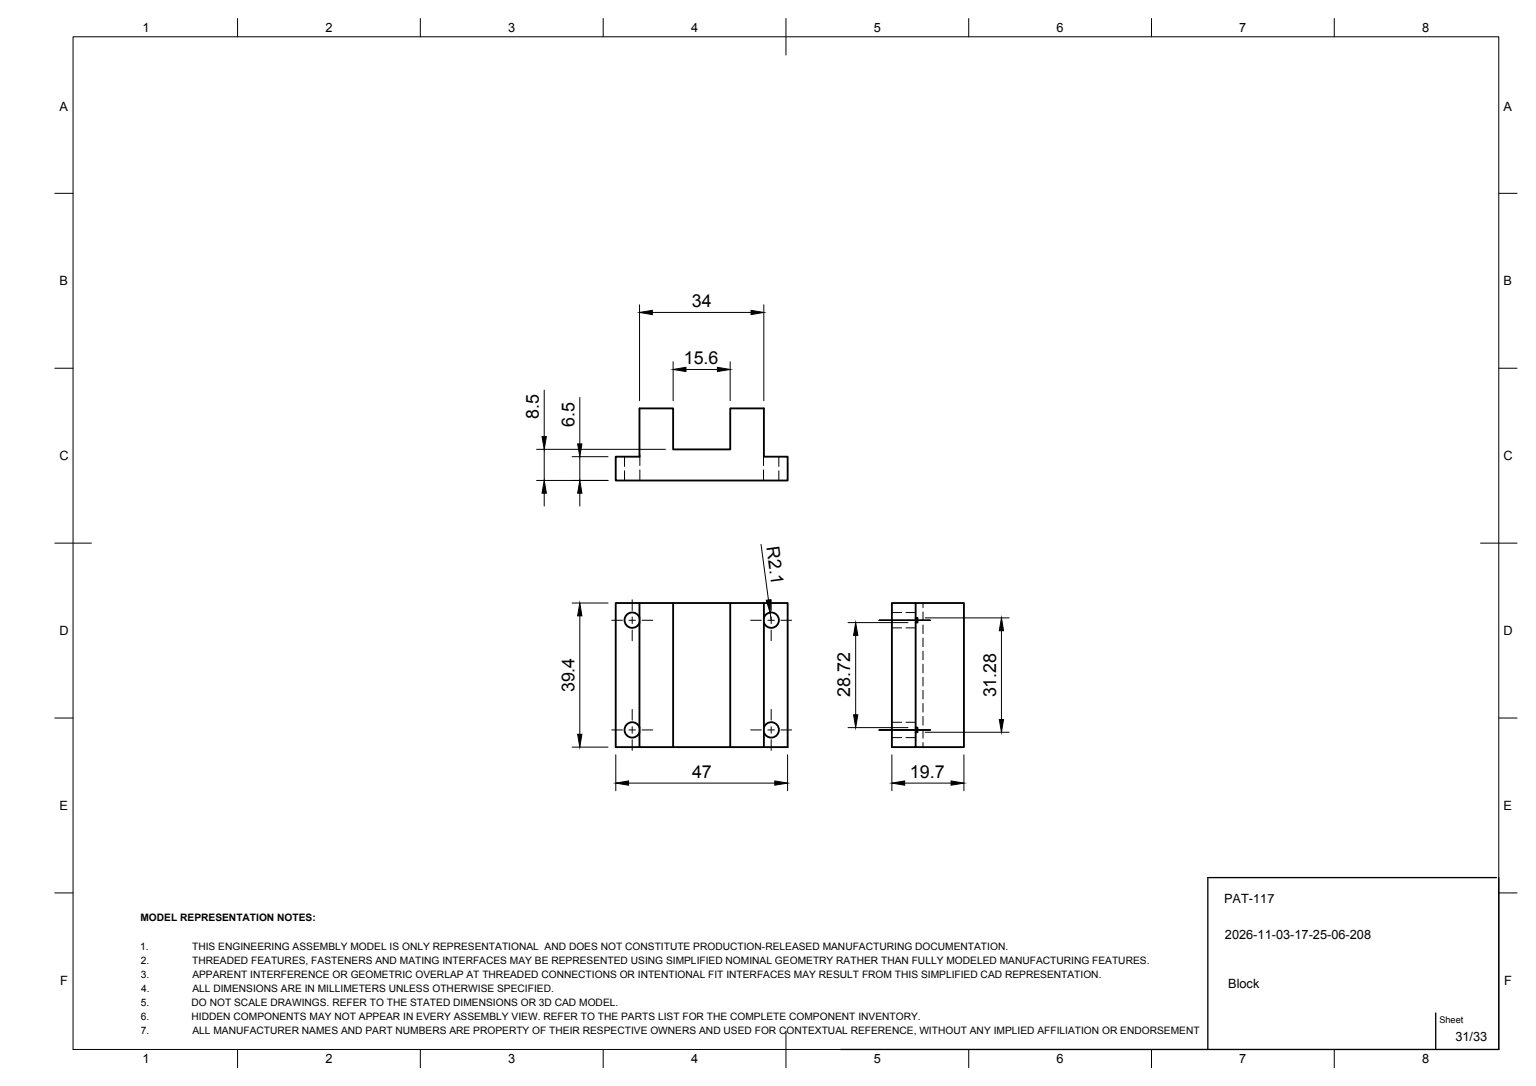
ISO-10303-21;
HEADER;
/* Generated by software containing ST-Developer
 * from STEP Tools, Inc. (www.steptools.com) 
 */

FILE_DESCRIPTION(
/* description */ ('Counterbalanced vertical column'),
/* implementation_level */ '2;1');

FILE_NAME(
/* name */ 'Block.step',
/* time_stamp */ '2026-10-29T16:47:22-07:00',
/* author */ (''),
/* organization */ (''),
/* preprocessor_version */ 'ST-DEVELOPER v20.2',
/* originating_system */ 'Autodesk Translation Framework v15.17.0.0',
/* authorisation */ '');

FILE_SCHEMA (('AUTOMOTIVE_DESIGN { 1 0 10303 214 3 1 1 }'));
ENDSEC;

DATA;
#10=MECHANICAL_DESIGN_GEOMETRIC_PRESENTATION_REPRESENTATION('',(#380),#15040);
#310=SHAPE_REPRESENTATION_RELATIONSHIP('SRR','None',#15216,#345);
#345=ADVANCED_BREP_SHAPE_REPRESENTATION('',(#413),#15035);
#380=STYLED_ITEM('',(#15436),#413);
#413=MANIFOLD_SOLID_BREP('Body1',#7105);
#525=FACE_BOUND('',#1684,.T.);
#526=FACE_BOUND('',#1685,.T.);
#527=FACE_BOUND('',#1686,.T.);
#528=FACE_BOUND('',#1687,.T.);
#766=PLANE('',#8052);
#767=PLANE('',#8058);
#768=PLANE('',#8064);
#769=PLANE('',#8070);
#770=PLANE('',#8076);
#771=PLANE('',#8077);
#772=PLANE('',#8078);
#773=PLANE('',#8079);
#774=PLANE('',#8080);
#775=PLANE('',#8081);
#776=PLANE('',#8082);
#777=PLANE('',#8083);
#778=PLANE('',#8084);
#779=PLANE('',#8085);
#780=PLANE('',#8086);
#781=PLANE('',#8087);
#782=PLANE('',#8088);
#783=PLANE('',#8089);
#1156=FACE_OUTER_BOUND('',#1670,.T.);
#1157=FACE_OUTER_BOUND('',#1671,.T.);
#1158=FACE_OUTER_BOUND('',#1672,.T.);
#1159=FACE_OUTER_BOUND('',#1673,.T.);
#1160=FACE_OUTER_BOUND('',#1674,.T.);
#1161=FACE_OUTER_BOUND('',#1675,.T.);
#1162=FACE_OUTER_BOUND('',#1676,.T.);
#1163=FACE_OUTER_BOUND('',#1677,.T.);
#1164=FACE_OUTER_BOUND('',#1678,.T.);
#1165=FACE_OUTER_BOUND('',#1679,.T.);
#1166=FACE_OUTER_BOUND('',#1680,.T.);
#1167=FACE_OUTER_BOUND('',#1681,.T.);
#1168=FACE_OUTER_BOUND('',#1682,.T.);
#1169=FACE_OUTER_BOUND('',#1683,.T.);
#1170=FACE_OUTER_BOUND('',#1688,.T.);
#1171=FACE_OUTER_BOUND('',#1689,.T.);
#1172=FACE_OUTER_BOUND('',#1690,.T.);
#1173=FACE_OUTER_BOUND('',#1691,.T.);
#1174=FACE_OUTER_BOUND('',#1692,.T.);
#1175=FACE_OUTER_BOUND('',#1693,.T.);
#1176=FACE_OUTER_BOUND('',#1694,.T.);
#1177=FACE_OUTER_BOUND('',#1695,.T.);
#1670=EDGE_LOOP('',(#6210,#6211));
#1671=EDGE_LOOP('',(#6212,#6213,#6214,#6215,#6216,#6217,#6218,#6219));
#1672=EDGE_LOOP('',(#6220,#6221));
#1673=EDGE_LOOP('',(#6222,#6223,#6224,#6225,#6226,#6227,#6228,#6229));
#1674=EDGE_LOOP('',(#6230,#6231));
#1675=EDGE_LOOP('',(#6232,#6233,#6234,#6235,#6236,#6237,#6238,#6239));
#1676=EDGE_LOOP('',(#6240,#6241));
#1677=EDGE_LOOP('',(#6242,#6243,#6244,#6245,#6246,#6247,#6248,#6249));
#1678=EDGE_LOOP('',(#6250,#6251,#6252,#6253,#6254,#6255,#6256,#6257,#6258,
#6259,#6260,#6261));
#1679=EDGE_LOOP('',(#6262,#6263,#6264,#6265,#6266,#6267,#6268,#6269,#6270,
#6271,#6272,#6273));
#1680=EDGE_LOOP('',(#6274,#6275,#6276,#6277,#6278,#6279,#6280,#6281,#6282,
#6283,#6284,#6285));
#1681=EDGE_LOOP('',(#6286,#6287,#6288,#6289,#6290,#6291,#6292,#6293,#6294,
#6295));
#1682=EDGE_LOOP('',(#6296,#6297,#6298,#6299));
#1683=EDGE_LOOP('',(#6300,#6301,#6302,#6303));
#1684=EDGE_LOOP('',(#6304));
#1685=EDGE_LOOP('',(#6305));
#1686=EDGE_LOOP('',(#6306));
#1687=EDGE_LOOP('',(#6307));
#1688=EDGE_LOOP('',(#6308,#6309,#6310,#6311));
#1689=EDGE_LOOP('',(#6312,#6313,#6314,#6315,#6316,#6317,#6318,#6319,#6320,
#6321));
#1690=EDGE_LOOP('',(#6322,#6323,#6324,#6325));
#1691=EDGE_LOOP('',(#6326,#6327,#6328,#6329));
#1692=EDGE_LOOP('',(#6330,#6331,#6332,#6333));
#1693=EDGE_LOOP('',(#6334,#6335,#6336,#6337));
#1694=EDGE_LOOP('',(#6338,#6339,#6340,#6341));
#1695=EDGE_LOOP('',(#6342,#6343,#6344,#6345,#6346,#6347,#6348,#6349,#6350,
#6351,#6352,#6353));
#2271=LINE('',#14525,#2942);
#2272=LINE('',#14529,#2943);
#2273=LINE('',#14533,#2944);
#2274=LINE('',#14537,#2945);
#2275=LINE('',#14541,#2946);
#2276=LINE('',#14545,#2947);
#2277=LINE('',#14549,#2948);
#2278=LINE('',#14553,#2949);
#2279=LINE('',#14557,#2950);
#2280=LINE('',#14561,#2951);
#2281=LINE('',#14565,#2952);
#2282=LINE('',#14569,#2953);
#2283=LINE('',#14573,#2954);
#2284=LINE('',#14577,#2955);
#2285=LINE('',#14581,#2956);
#2286=LINE('',#14585,#2957);
#2287=LINE('',#14587,#2958);
#2288=LINE('',#14589,#2959);
#2289=LINE('',#14591,#2960);
#2290=LINE('',#14593,#2961);
#2291=LINE('',#14595,#2962);
#2292=LINE('',#14596,#2963);
#2293=LINE('',#14598,#2964);
#2294=LINE('',#14600,#2965);
#2295=LINE('',#14602,#2966);
#2296=LINE('',#14604,#2967);
#2297=LINE('',#14606,#2968);
#2298=LINE('',#14607,#2969);
#2299=LINE('',#14610,#2970);
#2300=LINE('',#14612,#2971);
#2301=LINE('',#14614,#2972);
#2302=LINE('',#14616,#2973);
#2303=LINE('',#14617,#2974);
#2304=LINE('',#14619,#2975);
#2305=LINE('',#14621,#2976);
#2306=LINE('',#14623,#2977);
#2307=LINE('',#14625,#2978);
#2308=LINE('',#14626,#2979);
#2309=LINE('',#14629,#2980);
#2310=LINE('',#14630,#2981);
#2311=LINE('',#14633,#2982);
#2312=LINE('',#14634,#2983);
#2313=LINE('',#14637,#2984);
#2314=LINE('',#14638,#2985);
#2315=LINE('',#14641,#2986);
#2316=LINE('',#14642,#2987);
#2317=LINE('',#14644,#2988);
#2318=LINE('',#14647,#2989);
#2319=LINE('',#14648,#2990);
#2320=LINE('',#14651,#2991);
#2321=LINE('',#14652,#2992);
#2322=LINE('',#14655,#2993);
#2323=LINE('',#14656,#2994);
#2324=LINE('',#14659,#2995);
#2325=LINE('',#14660,#2996);
#2326=LINE('',#14662,#2997);
#2942=VECTOR('',#9851,1.);
#2943=VECTOR('',#9856,1.);
#2944=VECTOR('',#9859,0.21);
#2945=VECTOR('',#9864,1.);
#2946=VECTOR('',#9867,1.);
#2947=VECTOR('',#9872,1.);
#2948=VECTOR('',#9875,0.21);
#2949=VECTOR('',#9880,1.);
#2950=VECTOR('',#9883,1.);
#2951=VECTOR('',#9888,1.);
#2952=VECTOR('',#9891,0.21);
#2953=VECTOR('',#9896,1.);
#2954=VECTOR('',#9899,1.);
#2955=VECTOR('',#9904,1.);
#2956=VECTOR('',#9907,0.21);
#2957=VECTOR('',#9912,1.);
#2958=VECTOR('',#9915,1.);
#2959=VECTOR('',#9916,1.);
#2960=VECTOR('',#9917,1.);
#2961=VECTOR('',#9918,1.);
#2962=VECTOR('',#9919,1.);
#2963=VECTOR('',#9920,1.);
#2964=VECTOR('',#9923,1.);
#2965=VECTOR('',#9924,1.);
#2966=VECTOR('',#9925,1.);
#2967=VECTOR('',#9926,1.);
#2968=VECTOR('',#9927,1.);
#2969=VECTOR('',#9928,1.);
#2970=VECTOR('',#9931,1.);
#2971=VECTOR('',#9932,1.);
#2972=VECTOR('',#9933,1.);
#2973=VECTOR('',#9934,1.);
#2974=VECTOR('',#9935,1.);
#2975=VECTOR('',#9936,1.);
#2976=VECTOR('',#9937,1.);
#2977=VECTOR('',#9938,1.);
#2978=VECTOR('',#9939,1.);
#2979=VECTOR('',#9940,1.);
#2980=VECTOR('',#9943,1.);
#2981=VECTOR('',#9944,1.);
#2982=VECTOR('',#9947,1.);
#2983=VECTOR('',#9948,1.);
#2984=VECTOR('',#9951,1.);
#2985=VECTOR('',#9952,1.);
#2986=VECTOR('',#9955,1.);
#2987=VECTOR('',#9956,1.);
#2988=VECTOR('',#9959,1.);
#2989=VECTOR('',#9962,1.);
#2990=VECTOR('',#9963,1.);
#2991=VECTOR('',#9966,1.);
#2992=VECTOR('',#9967,1.);
#2993=VECTOR('',#9970,1.);
#2994=VECTOR('',#9971,1.);
#2995=VECTOR('',#9974,1.);
#2996=VECTOR('',#9975,1.);
#2997=VECTOR('',#9978,1.);
#3275=CIRCLE('',#8053,0.21);
#3276=CIRCLE('',#8055,0.21);
#3277=CIRCLE('',#8056,0.21);
#3278=CIRCLE('',#8057,0.21);
#3279=CIRCLE('',#8059,0.21);
#3280=CIRCLE('',#8061,0.21);
#3281=CIRCLE('',#8062,0.21);
#3282=CIRCLE('',#8063,0.21);
#3283=CIRCLE('',#8065,0.21);
#3284=CIRCLE('',#8067,0.21);
#3285=CIRCLE('',#8068,0.21);
#3286=CIRCLE('',#8069,0.21);
#3287=CIRCLE('',#8071,0.21);
#3288=CIRCLE('',#8073,0.21);
#3289=CIRCLE('',#8074,0.21);
#3290=CIRCLE('',#8075,0.21);
#3776=VERTEX_POINT('',#14523);
#3777=VERTEX_POINT('',#14524);
#3778=VERTEX_POINT('',#14528);
#3779=VERTEX_POINT('',#14530);
#3780=VERTEX_POINT('',#14532);
#3781=VERTEX_POINT('',#14535);
#3782=VERTEX_POINT('',#14539);
#3783=VERTEX_POINT('',#14540);
#3784=VERTEX_POINT('',#14544);
#3785=VERTEX_POINT('',#14546);
#3786=VERTEX_POINT('',#14548);
#3787=VERTEX_POINT('',#14551);
#3788=VERTEX_POINT('',#14555);
#3789=VERTEX_POINT('',#14556);
#3790=VERTEX_POINT('',#14560);
#3791=VERTEX_POINT('',#14562);
#3792=VERTEX_POINT('',#14564);
#3793=VERTEX_POINT('',#14567);
#3794=VERTEX_POINT('',#14571);
#3795=VERTEX_POINT('',#14572);
#3796=VERTEX_POINT('',#14576);
#3797=VERTEX_POINT('',#14578);
#3798=VERTEX_POINT('',#14580);
#3799=VERTEX_POINT('',#14583);
#3800=VERTEX_POINT('',#14588);
#3801=VERTEX_POINT('',#14590);
#3802=VERTEX_POINT('',#14592);
#3803=VERTEX_POINT('',#14594);
#3804=VERTEX_POINT('',#14599);
#3805=VERTEX_POINT('',#14601);
#3806=VERTEX_POINT('',#14603);
#3807=VERTEX_POINT('',#14605);
#3808=VERTEX_POINT('',#14609);
#3809=VERTEX_POINT('',#14611);
#3810=VERTEX_POINT('',#14613);
#3811=VERTEX_POINT('',#14615);
#3812=VERTEX_POINT('',#14618);
#3813=VERTEX_POINT('',#14620);
#3814=VERTEX_POINT('',#14622);
#3815=VERTEX_POINT('',#14624);
#3816=VERTEX_POINT('',#14628);
#3817=VERTEX_POINT('',#14632);
#3818=VERTEX_POINT('',#14636);
#3819=VERTEX_POINT('',#14640);
#3820=VERTEX_POINT('',#14646);
#3821=VERTEX_POINT('',#14650);
#3822=VERTEX_POINT('',#14654);
#3823=VERTEX_POINT('',#14658);
#4606=EDGE_CURVE('',#3776,#3777,#2271,.T.);
#4607=EDGE_CURVE('',#3776,#3777,#3275,.T.);
#4608=EDGE_CURVE('',#3778,#3776,#2272,.T.);
#4609=EDGE_CURVE('',#3779,#3778,#3276,.T.);
#4610=EDGE_CURVE('',#3779,#3780,#2273,.T.);
#4611=EDGE_CURVE('',#3780,#3780,#3277,.T.);
#4612=EDGE_CURVE('',#3781,#3779,#3278,.T.);
#4613=EDGE_CURVE('',#3777,#3781,#2274,.T.);
#4614=EDGE_CURVE('',#3782,#3783,#2275,.T.);
#4615=EDGE_CURVE('',#3782,#3783,#3279,.T.);
#4616=EDGE_CURVE('',#3784,#3782,#2276,.T.);
#4617=EDGE_CURVE('',#3785,#3784,#3280,.T.);
#4618=EDGE_CURVE('',#3785,#3786,#2277,.T.);
#4619=EDGE_CURVE('',#3786,#3786,#3281,.T.);
#4620=EDGE_CURVE('',#3787,#3785,#3282,.T.);
#4621=EDGE_CURVE('',#3783,#3787,#2278,.T.);
#4622=EDGE_CURVE('',#3788,#3789,#2279,.T.);
#4623=EDGE_CURVE('',#3788,#3789,#3283,.T.);
#4624=EDGE_CURVE('',#3790,#3788,#2280,.T.);
#4625=EDGE_CURVE('',#3791,#3790,#3284,.T.);
#4626=EDGE_CURVE('',#3791,#3792,#2281,.T.);
#4627=EDGE_CURVE('',#3792,#3792,#3285,.T.);
#4628=EDGE_CURVE('',#3793,#3791,#3286,.T.);
#4629=EDGE_CURVE('',#3789,#3793,#2282,.T.);
#4630=EDGE_CURVE('',#3794,#3795,#2283,.T.);
#4631=EDGE_CURVE('',#3794,#3795,#3287,.T.);
#4632=EDGE_CURVE('',#3796,#3794,#2284,.T.);
#4633=EDGE_CURVE('',#3797,#3796,#3288,.T.);
#4634=EDGE_CURVE('',#3797,#3798,#2285,.T.);
#4635=EDGE_CURVE('',#3798,#3798,#3289,.T.);
#4636=EDGE_CURVE('',#3799,#3797,#3290,.T.);
#4637=EDGE_CURVE('',#3795,#3799,#2286,.T.);
#4638=EDGE_CURVE('',#3781,#3790,#2287,.T.);
#4639=EDGE_CURVE('',#3793,#3800,#2288,.T.);
#4640=EDGE_CURVE('',#3801,#3800,#2289,.T.);
#4641=EDGE_CURVE('',#3801,#3802,#2290,.T.);
#4642=EDGE_CURVE('',#3803,#3802,#2291,.T.);
#4643=EDGE_CURVE('',#3803,#3778,#2292,.T.);
#4644=EDGE_CURVE('',#3787,#3796,#2293,.T.);
#4645=EDGE_CURVE('',#3799,#3804,#2294,.T.);
#4646=EDGE_CURVE('',#3805,#3804,#2295,.T.);
#4647=EDGE_CURVE('',#3806,#3805,#2296,.T.);
#4648=EDGE_CURVE('',#3807,#3806,#2297,.T.);
#4649=EDGE_CURVE('',#3807,#3784,#2298,.T.);
#4650=EDGE_CURVE('',#3800,#3808,#2299,.T.);
#4651=EDGE_CURVE('',#3808,#3809,#2300,.T.);
#4652=EDGE_CURVE('',#3809,#3810,#2301,.T.);
#4653=EDGE_CURVE('',#3810,#3811,#2302,.T.);
#4654=EDGE_CURVE('',#3811,#3807,#2303,.T.);
#4655=EDGE_CURVE('',#3806,#3812,#2304,.T.);
#4656=EDGE_CURVE('',#3812,#3813,#2305,.T.);
#4657=EDGE_CURVE('',#3813,#3814,#2306,.T.);
#4658=EDGE_CURVE('',#3814,#3815,#2307,.T.);
#4659=EDGE_CURVE('',#3815,#3801,#2308,.T.);
#4660=EDGE_CURVE('',#3816,#3803,#2309,.T.);
#4661=EDGE_CURVE('',#3808,#3816,#2310,.T.);
#4662=EDGE_CURVE('',#3817,#3816,#2311,.T.);
#4663=EDGE_CURVE('',#3809,#3817,#2312,.T.);
#4664=EDGE_CURVE('',#3818,#3817,#2313,.T.);
#4665=EDGE_CURVE('',#3810,#3818,#2314,.T.);
#4666=EDGE_CURVE('',#3819,#3818,#2315,.T.);
#4667=EDGE_CURVE('',#3811,#3819,#2316,.T.);
#4668=EDGE_CURVE('',#3804,#3819,#2317,.T.);
#4669=EDGE_CURVE('',#3820,#3805,#2318,.T.);
#4670=EDGE_CURVE('',#3812,#3820,#2319,.T.);
#4671=EDGE_CURVE('',#3821,#3820,#2320,.T.);
#4672=EDGE_CURVE('',#3813,#3821,#2321,.T.);
#4673=EDGE_CURVE('',#3822,#3821,#2322,.T.);
#4674=EDGE_CURVE('',#3814,#3822,#2323,.T.);
#4675=EDGE_CURVE('',#3823,#3822,#2324,.T.);
#4676=EDGE_CURVE('',#3815,#3823,#2325,.T.);
#4677=EDGE_CURVE('',#3802,#3823,#2326,.T.);
#6210=ORIENTED_EDGE('',*,*,#4606,.F.);
#6211=ORIENTED_EDGE('',*,*,#4607,.T.);
#6212=ORIENTED_EDGE('',*,*,#4608,.F.);
#6213=ORIENTED_EDGE('',*,*,#4609,.F.);
#6214=ORIENTED_EDGE('',*,*,#4610,.T.);
#6215=ORIENTED_EDGE('',*,*,#4611,.F.);
#6216=ORIENTED_EDGE('',*,*,#4610,.F.);
#6217=ORIENTED_EDGE('',*,*,#4612,.F.);
#6218=ORIENTED_EDGE('',*,*,#4613,.F.);
#6219=ORIENTED_EDGE('',*,*,#4607,.F.);
#6220=ORIENTED_EDGE('',*,*,#4614,.F.);
#6221=ORIENTED_EDGE('',*,*,#4615,.T.);
#6222=ORIENTED_EDGE('',*,*,#4616,.F.);
#6223=ORIENTED_EDGE('',*,*,#4617,.F.);
#6224=ORIENTED_EDGE('',*,*,#4618,.T.);
#6225=ORIENTED_EDGE('',*,*,#4619,.F.);
#6226=ORIENTED_EDGE('',*,*,#4618,.F.);
#6227=ORIENTED_EDGE('',*,*,#4620,.F.);
#6228=ORIENTED_EDGE('',*,*,#4621,.F.);
#6229=ORIENTED_EDGE('',*,*,#4615,.F.);
#6230=ORIENTED_EDGE('',*,*,#4622,.F.);
#6231=ORIENTED_EDGE('',*,*,#4623,.T.);
#6232=ORIENTED_EDGE('',*,*,#4624,.F.);
#6233=ORIENTED_EDGE('',*,*,#4625,.F.);
#6234=ORIENTED_EDGE('',*,*,#4626,.T.);
#6235=ORIENTED_EDGE('',*,*,#4627,.F.);
#6236=ORIENTED_EDGE('',*,*,#4626,.F.);
#6237=ORIENTED_EDGE('',*,*,#4628,.F.);
#6238=ORIENTED_EDGE('',*,*,#4629,.F.);
#6239=ORIENTED_EDGE('',*,*,#4623,.F.);
#6240=ORIENTED_EDGE('',*,*,#4630,.F.);
#6241=ORIENTED_EDGE('',*,*,#4631,.T.);
#6242=ORIENTED_EDGE('',*,*,#4632,.F.);
#6243=ORIENTED_EDGE('',*,*,#4633,.F.);
#6244=ORIENTED_EDGE('',*,*,#4634,.T.);
#6245=ORIENTED_EDGE('',*,*,#4635,.F.);
#6246=ORIENTED_EDGE('',*,*,#4634,.F.);
#6247=ORIENTED_EDGE('',*,*,#4636,.F.);
#6248=ORIENTED_EDGE('',*,*,#4637,.F.);
#6249=ORIENTED_EDGE('',*,*,#4631,.F.);
#6250=ORIENTED_EDGE('',*,*,#4608,.T.);
#6251=ORIENTED_EDGE('',*,*,#4606,.T.);
#6252=ORIENTED_EDGE('',*,*,#4613,.T.);
#6253=ORIENTED_EDGE('',*,*,#4638,.T.);
#6254=ORIENTED_EDGE('',*,*,#4624,.T.);
#6255=ORIENTED_EDGE('',*,*,#4622,.T.);
#6256=ORIENTED_EDGE('',*,*,#4629,.T.);
#6257=ORIENTED_EDGE('',*,*,#4639,.T.);
#6258=ORIENTED_EDGE('',*,*,#4640,.F.);
#6259=ORIENTED_EDGE('',*,*,#4641,.T.);
#6260=ORIENTED_EDGE('',*,*,#4642,.F.);
#6261=ORIENTED_EDGE('',*,*,#4643,.T.);
#6262=ORIENTED_EDGE('',*,*,#4616,.T.);
#6263=ORIENTED_EDGE('',*,*,#4614,.T.);
#6264=ORIENTED_EDGE('',*,*,#4621,.T.);
#6265=ORIENTED_EDGE('',*,*,#4644,.T.);
#6266=ORIENTED_EDGE('',*,*,#4632,.T.);
#6267=ORIENTED_EDGE('',*,*,#4630,.T.);
#6268=ORIENTED_EDGE('',*,*,#4637,.T.);
#6269=ORIENTED_EDGE('',*,*,#4645,.T.);
#6270=ORIENTED_EDGE('',*,*,#4646,.F.);
#6271=ORIENTED_EDGE('',*,*,#4647,.F.);
#6272=ORIENTED_EDGE('',*,*,#4648,.F.);
#6273=ORIENTED_EDGE('',*,*,#4649,.T.);
#6274=ORIENTED_EDGE('',*,*,#4640,.T.);
#6275=ORIENTED_EDGE('',*,*,#4650,.T.);
#6276=ORIENTED_EDGE('',*,*,#4651,.T.);
#6277=ORIENTED_EDGE('',*,*,#4652,.T.);
#6278=ORIENTED_EDGE('',*,*,#4653,.T.);
#6279=ORIENTED_EDGE('',*,*,#4654,.T.);
#6280=ORIENTED_EDGE('',*,*,#4648,.T.);
#6281=ORIENTED_EDGE('',*,*,#4655,.T.);
#6282=ORIENTED_EDGE('',*,*,#4656,.T.);
#6283=ORIENTED_EDGE('',*,*,#4657,.T.);
#6284=ORIENTED_EDGE('',*,*,#4658,.T.);
#6285=ORIENTED_EDGE('',*,*,#4659,.T.);
#6286=ORIENTED_EDGE('',*,*,#4612,.T.);
#6287=ORIENTED_EDGE('',*,*,#4609,.T.);
#6288=ORIENTED_EDGE('',*,*,#4643,.F.);
#6289=ORIENTED_EDGE('',*,*,#4660,.F.);
#6290=ORIENTED_EDGE('',*,*,#4661,.F.);
#6291=ORIENTED_EDGE('',*,*,#4650,.F.);
#6292=ORIENTED_EDGE('',*,*,#4639,.F.);
#6293=ORIENTED_EDGE('',*,*,#4628,.T.);
#6294=ORIENTED_EDGE('',*,*,#4625,.T.);
#6295=ORIENTED_EDGE('',*,*,#4638,.F.);
#6296=ORIENTED_EDGE('',*,*,#4661,.T.);
#6297=ORIENTED_EDGE('',*,*,#4662,.F.);
#6298=ORIENTED_EDGE('',*,*,#4663,.F.);
#6299=ORIENTED_EDGE('',*,*,#4651,.F.);
#6300=ORIENTED_EDGE('',*,*,#4663,.T.);
#6301=ORIENTED_EDGE('',*,*,#4664,.F.);
#6302=ORIENTED_EDGE('',*,*,#4665,.F.);
#6303=ORIENTED_EDGE('',*,*,#4652,.F.);
#6304=ORIENTED_EDGE('',*,*,#4611,.T.);
#6305=ORIENTED_EDGE('',*,*,#4619,.T.);
#6306=ORIENTED_EDGE('',*,*,#4627,.T.);
#6307=ORIENTED_EDGE('',*,*,#4635,.T.);
#6308=ORIENTED_EDGE('',*,*,#4665,.T.);
#6309=ORIENTED_EDGE('',*,*,#4666,.F.);
#6310=ORIENTED_EDGE('',*,*,#4667,.F.);
#6311=ORIENTED_EDGE('',*,*,#4653,.F.);
#6312=ORIENTED_EDGE('',*,*,#4620,.T.);
#6313=ORIENTED_EDGE('',*,*,#4617,.T.);
#6314=ORIENTED_EDGE('',*,*,#4649,.F.);
#6315=ORIENTED_EDGE('',*,*,#4654,.F.);
#6316=ORIENTED_EDGE('',*,*,#4667,.T.);
#6317=ORIENTED_EDGE('',*,*,#4668,.F.);
#6318=ORIENTED_EDGE('',*,*,#4645,.F.);
#6319=ORIENTED_EDGE('',*,*,#4636,.T.);
#6320=ORIENTED_EDGE('',*,*,#4633,.T.);
#6321=ORIENTED_EDGE('',*,*,#4644,.F.);
#6322=ORIENTED_EDGE('',*,*,#4647,.T.);
#6323=ORIENTED_EDGE('',*,*,#4669,.F.);
#6324=ORIENTED_EDGE('',*,*,#4670,.F.);
#6325=ORIENTED_EDGE('',*,*,#4655,.F.);
#6326=ORIENTED_EDGE('',*,*,#4670,.T.);
#6327=ORIENTED_EDGE('',*,*,#4671,.F.);
#6328=ORIENTED_EDGE('',*,*,#4672,.F.);
#6329=ORIENTED_EDGE('',*,*,#4656,.F.);
#6330=ORIENTED_EDGE('',*,*,#4672,.T.);
#6331=ORIENTED_EDGE('',*,*,#4673,.F.);
#6332=ORIENTED_EDGE('',*,*,#4674,.F.);
#6333=ORIENTED_EDGE('',*,*,#4657,.F.);
#6334=ORIENTED_EDGE('',*,*,#4674,.T.);
#6335=ORIENTED_EDGE('',*,*,#4675,.F.);
#6336=ORIENTED_EDGE('',*,*,#4676,.F.);
#6337=ORIENTED_EDGE('',*,*,#4658,.F.);
#6338=ORIENTED_EDGE('',*,*,#4676,.T.);
#6339=ORIENTED_EDGE('',*,*,#4677,.F.);
#6340=ORIENTED_EDGE('',*,*,#4641,.F.);
#6341=ORIENTED_EDGE('',*,*,#4659,.F.);
#6342=ORIENTED_EDGE('',*,*,#4642,.T.);
#6343=ORIENTED_EDGE('',*,*,#4677,.T.);
#6344=ORIENTED_EDGE('',*,*,#4675,.T.);
#6345=ORIENTED_EDGE('',*,*,#4673,.T.);
#6346=ORIENTED_EDGE('',*,*,#4671,.T.);
#6347=ORIENTED_EDGE('',*,*,#4669,.T.);
#6348=ORIENTED_EDGE('',*,*,#4646,.T.);
#6349=ORIENTED_EDGE('',*,*,#4668,.T.);
#6350=ORIENTED_EDGE('',*,*,#4666,.T.);
#6351=ORIENTED_EDGE('',*,*,#4664,.T.);
#6352=ORIENTED_EDGE('',*,*,#4662,.T.);
#6353=ORIENTED_EDGE('',*,*,#4660,.T.);
#6660=CYLINDRICAL_SURFACE('',#8054,0.21);
#6661=CYLINDRICAL_SURFACE('',#8060,0.21);
#6662=CYLINDRICAL_SURFACE('',#8066,0.21);
#6663=CYLINDRICAL_SURFACE('',#8072,0.21);
#6998=ADVANCED_FACE('',(#1156),#766,.T.);
#6999=ADVANCED_FACE('',(#1157),#6660,.F.);
#7000=ADVANCED_FACE('',(#1158),#767,.T.);
#7001=ADVANCED_FACE('',(#1159),#6661,.F.);
#7002=ADVANCED_FACE('',(#1160),#768,.T.);
#7003=ADVANCED_FACE('',(#1161),#6662,.F.);
#7004=ADVANCED_FACE('',(#1162),#769,.T.);
#7005=ADVANCED_FACE('',(#1163),#6663,.F.);
#7006=ADVANCED_FACE('',(#1164),#770,.T.);
#7007=ADVANCED_FACE('',(#1165),#771,.T.);
#7008=ADVANCED_FACE('',(#1166),#772,.T.);
#7009=ADVANCED_FACE('',(#1167),#773,.T.);
#7010=ADVANCED_FACE('',(#1168),#774,.T.);
#7011=ADVANCED_FACE('',(#1169,#525,#526,#527,#528),#775,.T.);
#7012=ADVANCED_FACE('',(#1170),#776,.T.);
#7013=ADVANCED_FACE('',(#1171),#777,.T.);
#7014=ADVANCED_FACE('',(#1172),#778,.T.);
#7015=ADVANCED_FACE('',(#1173),#779,.T.);
#7016=ADVANCED_FACE('',(#1174),#780,.T.);
#7017=ADVANCED_FACE('',(#1175),#781,.T.);
#7018=ADVANCED_FACE('',(#1176),#782,.T.);
#7019=ADVANCED_FACE('',(#1177),#783,.T.);
#7105=CLOSED_SHELL('',(#6998,#6999,#7000,#7001,#7002,#7003,#7004,#7005,
#7006,#7007,#7008,#7009,#7010,#7011,#7012,#7013,#7014,#7015,#7016,#7017,
#7018,#7019));
#8051=AXIS2_PLACEMENT_3D('',#14521,#9847,#9848);
#8052=AXIS2_PLACEMENT_3D('',#14522,#9849,#9850);
#8053=AXIS2_PLACEMENT_3D('',#14526,#9852,#9853);
#8054=AXIS2_PLACEMENT_3D('',#14527,#9854,#9855);
#8055=AXIS2_PLACEMENT_3D('',#14531,#9857,#9858);
#8056=AXIS2_PLACEMENT_3D('',#14534,#9860,#9861);
#8057=AXIS2_PLACEMENT_3D('',#14536,#9862,#9863);
#8058=AXIS2_PLACEMENT_3D('',#14538,#9865,#9866);
#8059=AXIS2_PLACEMENT_3D('',#14542,#9868,#9869);
#8060=AXIS2_PLACEMENT_3D('',#14543,#9870,#9871);
#8061=AXIS2_PLACEMENT_3D('',#14547,#9873,#9874);
#8062=AXIS2_PLACEMENT_3D('',#14550,#9876,#9877);
#8063=AXIS2_PLACEMENT_3D('',#14552,#9878,#9879);
#8064=AXIS2_PLACEMENT_3D('',#14554,#9881,#9882);
#8065=AXIS2_PLACEMENT_3D('',#14558,#9884,#9885);
#8066=AXIS2_PLACEMENT_3D('',#14559,#9886,#9887);
#8067=AXIS2_PLACEMENT_3D('',#14563,#9889,#9890);
#8068=AXIS2_PLACEMENT_3D('',#14566,#9892,#9893);
#8069=AXIS2_PLACEMENT_3D('',#14568,#9894,#9895);
#8070=AXIS2_PLACEMENT_3D('',#14570,#9897,#9898);
#8071=AXIS2_PLACEMENT_3D('',#14574,#9900,#9901);
#8072=AXIS2_PLACEMENT_3D('',#14575,#9902,#9903);
#8073=AXIS2_PLACEMENT_3D('',#14579,#9905,#9906);
#8074=AXIS2_PLACEMENT_3D('',#14582,#9908,#9909);
#8075=AXIS2_PLACEMENT_3D('',#14584,#9910,#9911);
#8076=AXIS2_PLACEMENT_3D('',#14586,#9913,#9914);
#8077=AXIS2_PLACEMENT_3D('',#14597,#9921,#9922);
#8078=AXIS2_PLACEMENT_3D('',#14608,#9929,#9930);
#8079=AXIS2_PLACEMENT_3D('',#14627,#9941,#9942);
#8080=AXIS2_PLACEMENT_3D('',#14631,#9945,#9946);
#8081=AXIS2_PLACEMENT_3D('',#14635,#9949,#9950);
#8082=AXIS2_PLACEMENT_3D('',#14639,#9953,#9954);
#8083=AXIS2_PLACEMENT_3D('',#14643,#9957,#9958);
#8084=AXIS2_PLACEMENT_3D('',#14645,#9960,#9961);
#8085=AXIS2_PLACEMENT_3D('',#14649,#9964,#9965);
#8086=AXIS2_PLACEMENT_3D('',#14653,#9968,#9969);
#8087=AXIS2_PLACEMENT_3D('',#14657,#9972,#9973);
#8088=AXIS2_PLACEMENT_3D('',#14661,#9976,#9977);
#8089=AXIS2_PLACEMENT_3D('',#14663,#9979,#9980);
#9847=DIRECTION('axis',(0.,0.,1.));
#9848=DIRECTION('refdir',(1.,0.,0.));
#9849=DIRECTION('center_axis',(0.,0.,1.));
#9850=DIRECTION('ref_axis',(1.,0.,0.));
#9851=DIRECTION('',(-1.,0.,0.));
#9852=DIRECTION('center_axis',(0.,0.,1.));
#9853=DIRECTION('ref_axis',(1.,0.,0.));
#9854=DIRECTION('center_axis',(0.,0.,1.));
#9855=DIRECTION('ref_axis',(1.,0.,0.));
#9856=DIRECTION('',(0.,0.,-1.));
#9857=DIRECTION('center_axis',(0.,0.,1.));
#9858=DIRECTION('ref_axis',(1.,0.,0.));
#9859=DIRECTION('',(0.,0.,1.));
#9860=DIRECTION('center_axis',(0.,0.,-1.));
#9861=DIRECTION('ref_axis',(1.,0.,0.));
#9862=DIRECTION('center_axis',(0.,0.,1.));
#9863=DIRECTION('ref_axis',(1.,0.,0.));
#9864=DIRECTION('',(0.,0.,1.));
#9865=DIRECTION('center_axis',(0.,0.,1.));
#9866=DIRECTION('ref_axis',(1.,0.,0.));
#9867=DIRECTION('',(1.,0.,0.));
#9868=DIRECTION('center_axis',(0.,0.,1.));
#9869=DIRECTION('ref_axis',(1.,0.,0.));
#9870=DIRECTION('center_axis',(0.,0.,1.));
#9871=DIRECTION('ref_axis',(1.,0.,0.));
#9872=DIRECTION('',(0.,0.,-1.));
#9873=DIRECTION('center_axis',(0.,0.,1.));
#9874=DIRECTION('ref_axis',(1.,0.,0.));
#9875=DIRECTION('',(0.,0.,1.));
#9876=DIRECTION('center_axis',(0.,0.,-1.));
#9877=DIRECTION('ref_axis',(1.,0.,0.));
#9878=DIRECTION('center_axis',(0.,0.,1.));
#9879=DIRECTION('ref_axis',(1.,0.,0.));
#9880=DIRECTION('',(0.,0.,1.));
#9881=DIRECTION('center_axis',(0.,0.,1.));
#9882=DIRECTION('ref_axis',(1.,0.,0.));
#9883=DIRECTION('',(-1.,0.,0.));
#9884=DIRECTION('center_axis',(0.,0.,1.));
#9885=DIRECTION('ref_axis',(1.,0.,0.));
#9886=DIRECTION('center_axis',(0.,0.,1.));
#9887=DIRECTION('ref_axis',(1.,0.,0.));
#9888=DIRECTION('',(0.,0.,-1.));
#9889=DIRECTION('center_axis',(0.,0.,1.));
#9890=DIRECTION('ref_axis',(1.,0.,0.));
#9891=DIRECTION('',(0.,0.,1.));
#9892=DIRECTION('center_axis',(0.,0.,-1.));
#9893=DIRECTION('ref_axis',(1.,0.,0.));
#9894=DIRECTION('center_axis',(0.,0.,1.));
#9895=DIRECTION('ref_axis',(1.,0.,0.));
#9896=DIRECTION('',(0.,0.,1.));
#9897=DIRECTION('center_axis',(0.,0.,1.));
#9898=DIRECTION('ref_axis',(1.,0.,0.));
#9899=DIRECTION('',(1.,0.,0.));
#9900=DIRECTION('center_axis',(0.,0.,1.));
#9901=DIRECTION('ref_axis',(1.,0.,0.));
#9902=DIRECTION('center_axis',(0.,0.,1.));
#9903=DIRECTION('ref_axis',(1.,0.,0.));
#9904=DIRECTION('',(0.,0.,-1.));
#9905=DIRECTION('center_axis',(0.,0.,1.));
#9906=DIRECTION('ref_axis',(1.,0.,0.));
#9907=DIRECTION('',(0.,0.,1.));
#9908=DIRECTION('center_axis',(0.,0.,-1.));
#9909=DIRECTION('ref_axis',(1.,0.,0.));
#9910=DIRECTION('center_axis',(0.,0.,1.));
#9911=DIRECTION('ref_axis',(1.,0.,0.));
#9912=DIRECTION('',(0.,0.,1.));
#9913=DIRECTION('center_axis',(0.,-1.,0.));
#9914=DIRECTION('ref_axis',(0.,0.,-1.));
#9915=DIRECTION('',(-1.,0.,0.));
#9916=DIRECTION('',(-1.,0.,0.));
#9917=DIRECTION('',(0.,0.,1.));
#9918=DIRECTION('',(1.,0.,0.));
#9919=DIRECTION('',(0.,0.,-1.));
#9920=DIRECTION('',(-1.,0.,0.));
#9921=DIRECTION('center_axis',(0.,1.,0.));
#9922=DIRECTION('ref_axis',(0.,0.,1.));
#9923=DIRECTION('',(1.,0.,0.));
#9924=DIRECTION('',(1.,0.,0.));
#9925=DIRECTION('',(0.,0.,1.));
#9926=DIRECTION('',(1.,0.,0.));
#9927=DIRECTION('',(0.,0.,-1.));
#9928=DIRECTION('',(1.,0.,0.));
#9929=DIRECTION('center_axis',(-1.,0.,0.));
#9930=DIRECTION('ref_axis',(0.,0.,1.));
#9931=DIRECTION('',(0.,-1.,0.));
#9932=DIRECTION('',(0.,0.,1.));
#9933=DIRECTION('',(0.,1.,0.));
#9934=DIRECTION('',(0.,0.,-1.));
#9935=DIRECTION('',(0.,-1.,0.));
#9936=DIRECTION('',(0.,-1.,0.));
#9937=DIRECTION('',(0.,0.,1.));
#9938=DIRECTION('',(0.,-1.,0.));
#9939=DIRECTION('',(0.,0.,-1.));
#9940=DIRECTION('',(0.,-1.,0.));
#9941=DIRECTION('center_axis',(0.,0.,-1.));
#9942=DIRECTION('ref_axis',(0.,1.,0.));
#9943=DIRECTION('',(0.,1.,0.));
#9944=DIRECTION('',(1.,0.,0.));
#9945=DIRECTION('center_axis',(0.,-1.,0.));
#9946=DIRECTION('ref_axis',(0.,0.,-1.));
#9947=DIRECTION('',(0.,0.,-1.));
#9948=DIRECTION('',(1.,0.,0.));
#9949=DIRECTION('center_axis',(0.,0.,1.));
#9950=DIRECTION('ref_axis',(0.,-1.,0.));
#9951=DIRECTION('',(0.,-1.,0.));
#9952=DIRECTION('',(1.,0.,0.));
#9953=DIRECTION('center_axis',(0.,1.,0.));
#9954=DIRECTION('ref_axis',(0.,0.,1.));
#9955=DIRECTION('',(0.,0.,1.));
#9956=DIRECTION('',(1.,0.,0.));
#9957=DIRECTION('center_axis',(0.,0.,-1.));
#9958=DIRECTION('ref_axis',(0.,1.,0.));
#9959=DIRECTION('',(0.,1.,0.));
#9960=DIRECTION('center_axis',(0.,0.,-1.));
#9961=DIRECTION('ref_axis',(0.,1.,0.));
#9962=DIRECTION('',(0.,1.,0.));
#9963=DIRECTION('',(1.,0.,0.));
#9964=DIRECTION('center_axis',(0.,-1.,0.));
#9965=DIRECTION('ref_axis',(0.,0.,-1.));
#9966=DIRECTION('',(0.,0.,-1.));
#9967=DIRECTION('',(1.,0.,0.));
#9968=DIRECTION('center_axis',(0.,0.,-1.));
#9969=DIRECTION('ref_axis',(0.,1.,0.));
#9970=DIRECTION('',(0.,1.,0.));
#9971=DIRECTION('',(1.,0.,0.));
#9972=DIRECTION('center_axis',(0.,1.,0.));
#9973=DIRECTION('ref_axis',(0.,0.,1.));
#9974=DIRECTION('',(0.,0.,1.));
#9975=DIRECTION('',(1.,0.,0.));
#9976=DIRECTION('center_axis',(0.,0.,-1.));
#9977=DIRECTION('ref_axis',(0.,1.,0.));
#9978=DIRECTION('',(0.,1.,0.));
#9979=DIRECTION('center_axis',(1.,0.,0.));
#9980=DIRECTION('ref_axis',(0.,0.,-1.));
#14521=CARTESIAN_POINT('',(0.,0.,0.));
#14522=CARTESIAN_POINT('Origin',(1.5,-1.9,1.7));
#14523=CARTESIAN_POINT('',(1.56403124237433,-1.7,1.7));
#14524=CARTESIAN_POINT('',(1.43596875762567,-1.7,1.7));
#14525=CARTESIAN_POINT('',(0.75,-1.7,1.7));
#14526=CARTESIAN_POINT('Origin',(1.5,-1.9,1.7));
#14527=CARTESIAN_POINT('Origin',(1.5,-1.9,1.7));
#14528=CARTESIAN_POINT('',(1.56403124237433,-1.7,1.75));
#14529=CARTESIAN_POINT('',(1.56403124237433,-1.7,1.7));
#14530=CARTESIAN_POINT('',(1.29,-1.9,1.75));
#14531=CARTESIAN_POINT('Origin',(1.5,-1.9,1.75));
#14532=CARTESIAN_POINT('',(1.29,-1.9,2.4));
#14533=CARTESIAN_POINT('',(1.29,-1.9,1.7));
#14534=CARTESIAN_POINT('Origin',(1.5,-1.9,2.4));
#14535=CARTESIAN_POINT('',(1.43596875762567,-1.7,1.75));
#14536=CARTESIAN_POINT('Origin',(1.5,-1.9,1.75));
#14537=CARTESIAN_POINT('',(1.43596875762567,-1.7,1.7));
#14538=CARTESIAN_POINT('Origin',(-1.5,1.9,1.7));
#14539=CARTESIAN_POINT('',(-1.56403124237433,1.7,1.7));
#14540=CARTESIAN_POINT('',(-1.43596875762567,1.7,1.7));
#14541=CARTESIAN_POINT('',(-0.75,1.7,1.7));
#14542=CARTESIAN_POINT('Origin',(-1.5,1.9,1.7));
#14543=CARTESIAN_POINT('Origin',(-1.5,1.9,1.7));
#14544=CARTESIAN_POINT('',(-1.56403124237433,1.7,1.75));
#14545=CARTESIAN_POINT('',(-1.56403124237433,1.7,1.7));
#14546=CARTESIAN_POINT('',(-1.71,1.9,1.75));
#14547=CARTESIAN_POINT('Origin',(-1.5,1.9,1.75));
#14548=CARTESIAN_POINT('',(-1.71,1.9,2.4));
#14549=CARTESIAN_POINT('',(-1.71,1.9,1.7));
#14550=CARTESIAN_POINT('Origin',(-1.5,1.9,2.4));
#14551=CARTESIAN_POINT('',(-1.43596875762567,1.7,1.75));
#14552=CARTESIAN_POINT('Origin',(-1.5,1.9,1.75));
#14553=CARTESIAN_POINT('',(-1.43596875762567,1.7,1.7));
#14554=CARTESIAN_POINT('Origin',(-1.5,-1.9,1.7));
#14555=CARTESIAN_POINT('',(-1.43596875762567,-1.7,1.7));
#14556=CARTESIAN_POINT('',(-1.56403124237433,-1.7,1.7));
#14557=CARTESIAN_POINT('',(-0.75,-1.7,1.7));
#14558=CARTESIAN_POINT('Origin',(-1.5,-1.9,1.7));
#14559=CARTESIAN_POINT('Origin',(-1.5,-1.9,1.7));
#14560=CARTESIAN_POINT('',(-1.43596875762567,-1.7,1.75));
#14561=CARTESIAN_POINT('',(-1.43596875762567,-1.7,1.7));
#14562=CARTESIAN_POINT('',(-1.71,-1.9,1.75));
#14563=CARTESIAN_POINT('Origin',(-1.5,-1.9,1.75));
#14564=CARTESIAN_POINT('',(-1.71,-1.9,2.4));
#14565=CARTESIAN_POINT('',(-1.71,-1.9,1.7));
#14566=CARTESIAN_POINT('Origin',(-1.5,-1.9,2.4));
#14567=CARTESIAN_POINT('',(-1.56403124237433,-1.7,1.75));
#14568=CARTESIAN_POINT('Origin',(-1.5,-1.9,1.75));
#14569=CARTESIAN_POINT('',(-1.56403124237433,-1.7,1.7));
#14570=CARTESIAN_POINT('Origin',(1.5,1.9,1.7));
#14571=CARTESIAN_POINT('',(1.43596875762567,1.7,1.7));
#14572=CARTESIAN_POINT('',(1.56403124237433,1.7,1.7));
#14573=CARTESIAN_POINT('',(0.75,1.7,1.7));
#14574=CARTESIAN_POINT('Origin',(1.5,1.9,1.7));
#14575=CARTESIAN_POINT('Origin',(1.5,1.9,1.7));
#14576=CARTESIAN_POINT('',(1.43596875762567,1.7,1.75));
#14577=CARTESIAN_POINT('',(1.43596875762567,1.7,1.7));
#14578=CARTESIAN_POINT('',(1.29,1.9,1.75));
#14579=CARTESIAN_POINT('Origin',(1.5,1.9,1.75));
#14580=CARTESIAN_POINT('',(1.29,1.9,2.4));
#14581=CARTESIAN_POINT('',(1.29,1.9,1.7));
#14582=CARTESIAN_POINT('Origin',(1.5,1.9,2.4));
#14583=CARTESIAN_POINT('',(1.56403124237433,1.7,1.75));
#14584=CARTESIAN_POINT('Origin',(1.5,1.9,1.75));
#14585=CARTESIAN_POINT('',(1.56403124237433,1.7,1.7));
#14586=CARTESIAN_POINT('Origin',(0.,-1.7,1.75));
#14587=CARTESIAN_POINT('',(0.,-1.7,1.75));
#14588=CARTESIAN_POINT('',(-1.97,-1.7,1.75));
#14589=CARTESIAN_POINT('',(0.,-1.7,1.75));
#14590=CARTESIAN_POINT('',(-1.97,-1.7,0.43));
#14591=CARTESIAN_POINT('',(-1.97,-1.7,1.75));
#14592=CARTESIAN_POINT('',(1.97,-1.7,0.43));
#14593=CARTESIAN_POINT('',(0.,-1.7,0.43));
#14594=CARTESIAN_POINT('',(1.97,-1.7,1.75));
#14595=CARTESIAN_POINT('',(1.97,-1.7,1.75));
#14596=CARTESIAN_POINT('',(0.,-1.7,1.75));
#14597=CARTESIAN_POINT('Origin',(0.,1.7,0.43));
#14598=CARTESIAN_POINT('',(0.,1.7,1.75));
#14599=CARTESIAN_POINT('',(1.97,1.7,1.75));
#14600=CARTESIAN_POINT('',(0.,1.7,1.75));
#14601=CARTESIAN_POINT('',(1.97,1.7,0.43));
#14602=CARTESIAN_POINT('',(1.97,1.7,0.43));
#14603=CARTESIAN_POINT('',(-1.97,1.7,0.43));
#14604=CARTESIAN_POINT('',(0.,1.7,0.43));
#14605=CARTESIAN_POINT('',(-1.97,1.7,1.75));
#14606=CARTESIAN_POINT('',(-1.97,1.7,0.43));
#14607=CARTESIAN_POINT('',(0.,1.7,1.75));
#14608=CARTESIAN_POINT('Origin',(-1.97,0.,1.415));
#14609=CARTESIAN_POINT('',(-1.97,-2.35,1.75));
#14610=CARTESIAN_POINT('',(-1.97,-2.35,1.75));
#14611=CARTESIAN_POINT('',(-1.97,-2.35,2.4));
#14612=CARTESIAN_POINT('',(-1.97,-2.35,2.4));
#14613=CARTESIAN_POINT('',(-1.97,2.35,2.4));
#14614=CARTESIAN_POINT('',(-1.97,2.35,2.4));
#14615=CARTESIAN_POINT('',(-1.97,2.35,1.75));
#14616=CARTESIAN_POINT('',(-1.97,2.35,1.75));
#14617=CARTESIAN_POINT('',(-1.97,1.7,1.75));
#14618=CARTESIAN_POINT('',(-1.97,0.78,0.43));
#14619=CARTESIAN_POINT('',(-1.97,0.78,0.43));
#14620=CARTESIAN_POINT('',(-1.97,0.78,1.55));
#14621=CARTESIAN_POINT('',(-1.97,0.78,1.55));
#14622=CARTESIAN_POINT('',(-1.97,-0.78,1.55));
#14623=CARTESIAN_POINT('',(-1.97,-0.78,1.55));
#14624=CARTESIAN_POINT('',(-1.97,-0.78,0.43));
#14625=CARTESIAN_POINT('',(-1.97,-0.78,0.43));
#14626=CARTESIAN_POINT('',(-1.97,-1.7,0.43));
#14627=CARTESIAN_POINT('Origin',(0.,-2.35,1.75));
#14628=CARTESIAN_POINT('',(1.97,-2.35,1.75));
#14629=CARTESIAN_POINT('',(1.97,-2.35,1.75));
#14630=CARTESIAN_POINT('',(0.,-2.35,1.75));
#14631=CARTESIAN_POINT('Origin',(0.,-2.35,2.4));
#14632=CARTESIAN_POINT('',(1.97,-2.35,2.4));
#14633=CARTESIAN_POINT('',(1.97,-2.35,2.4));
#14634=CARTESIAN_POINT('',(0.,-2.35,2.4));
#14635=CARTESIAN_POINT('Origin',(0.,2.35,2.4));
#14636=CARTESIAN_POINT('',(1.97,2.35,2.4));
#14637=CARTESIAN_POINT('',(1.97,2.35,2.4));
#14638=CARTESIAN_POINT('',(0.,2.35,2.4));
#14639=CARTESIAN_POINT('Origin',(0.,2.35,1.75));
#14640=CARTESIAN_POINT('',(1.97,2.35,1.75));
#14641=CARTESIAN_POINT('',(1.97,2.35,1.75));
#14642=CARTESIAN_POINT('',(0.,2.35,1.75));
#14643=CARTESIAN_POINT('Origin',(0.,1.7,1.75));
#14644=CARTESIAN_POINT('',(1.97,1.7,1.75));
#14645=CARTESIAN_POINT('Origin',(0.,0.78,0.43));
#14646=CARTESIAN_POINT('',(1.97,0.78,0.43));
#14647=CARTESIAN_POINT('',(1.97,0.78,0.43));
#14648=CARTESIAN_POINT('',(0.,0.78,0.43));
#14649=CARTESIAN_POINT('Origin',(0.,0.78,1.55));
#14650=CARTESIAN_POINT('',(1.97,0.78,1.55));
#14651=CARTESIAN_POINT('',(1.97,0.78,1.55));
#14652=CARTESIAN_POINT('',(0.,0.78,1.55));
#14653=CARTESIAN_POINT('Origin',(0.,-0.78,1.55));
#14654=CARTESIAN_POINT('',(1.97,-0.78,1.55));
#14655=CARTESIAN_POINT('',(1.97,-0.78,1.55));
#14656=CARTESIAN_POINT('',(0.,-0.78,1.55));
#14657=CARTESIAN_POINT('Origin',(0.,-0.78,0.43));
#14658=CARTESIAN_POINT('',(1.97,-0.78,0.43));
#14659=CARTESIAN_POINT('',(1.97,-0.78,0.43));
#14660=CARTESIAN_POINT('',(0.,-0.78,0.43));
#14661=CARTESIAN_POINT('Origin',(0.,-1.7,0.43));
#14662=CARTESIAN_POINT('',(1.97,-1.7,0.43));
#14663=CARTESIAN_POINT('Origin',(1.97,0.,1.415));
#14995=UNCERTAINTY_MEASURE_WITH_UNIT(LENGTH_MEASURE(0.001),#15041,
'DISTANCE_ACCURACY_VALUE',
'Maximum model space distance between geometric entities at asserted c
onnectivities');
#15000=UNCERTAINTY_MEASURE_WITH_UNIT(LENGTH_MEASURE(0.001),#15041,
'DISTANCE_ACCURACY_VALUE',
'Maximum model space distance between geometric entities at asserted c
onnectivities');
#15035=(
GEOMETRIC_REPRESENTATION_CONTEXT(3)
GLOBAL_UNCERTAINTY_ASSIGNED_CONTEXT((#14995))
GLOBAL_UNIT_ASSIGNED_CONTEXT((#15041,#15043,#15044))
REPRESENTATION_CONTEXT('','3D')
);
#15040=(
GEOMETRIC_REPRESENTATION_CONTEXT(3)
GLOBAL_UNCERTAINTY_ASSIGNED_CONTEXT((#15000))
GLOBAL_UNIT_ASSIGNED_CONTEXT((#15041,#15043,#15044))
REPRESENTATION_CONTEXT('','3D')
);
#15041=(
LENGTH_UNIT()
NAMED_UNIT(*)
SI_UNIT(.CENTI.,.METRE.)
);
#15043=(
NAMED_UNIT(*)
PLANE_ANGLE_UNIT()
SI_UNIT($,.RADIAN.)
);
#15044=(
NAMED_UNIT(*)
SI_UNIT($,.STERADIAN.)
SOLID_ANGLE_UNIT()
);
#15079=SHAPE_DEFINITION_REPRESENTATION(#15118,#15216);
#15118=PRODUCT_DEFINITION_SHAPE('',$,#15256);
#15216=SHAPE_REPRESENTATION('',(#8051),#15035);
#15221=PRODUCT_DEFINITION_CONTEXT('part definition',#15340,'design');
#15256=PRODUCT_DEFINITION('Block','Block',#15295,#15221);
#15295=PRODUCT_DEFINITION_FORMATION('',$,#15376);
#15340=APPLICATION_CONTEXT(
'Core Data for Automotive Mechanical Design Process');
#15341=PRODUCT_CONTEXT('part definition',#15340,'mechanical');
#15376=PRODUCT('Block','Block','Block',(#15341));
#15430=COLOUR_RGB('Dark Blue',0.08,0.2,0.34);
#15431=FILL_AREA_STYLE_COLOUR('',#15430);
#15432=FILL_AREA_STYLE('',(#15431));
#15433=SURFACE_STYLE_FILL_AREA(#15432);
#15434=SURFACE_SIDE_STYLE('',(#15433));
#15435=SURFACE_STYLE_USAGE(.BOTH.,#15434);
#15436=PRESENTATION_STYLE_ASSIGNMENT((#15435));
ENDSEC;
END-ISO-10303-21;
